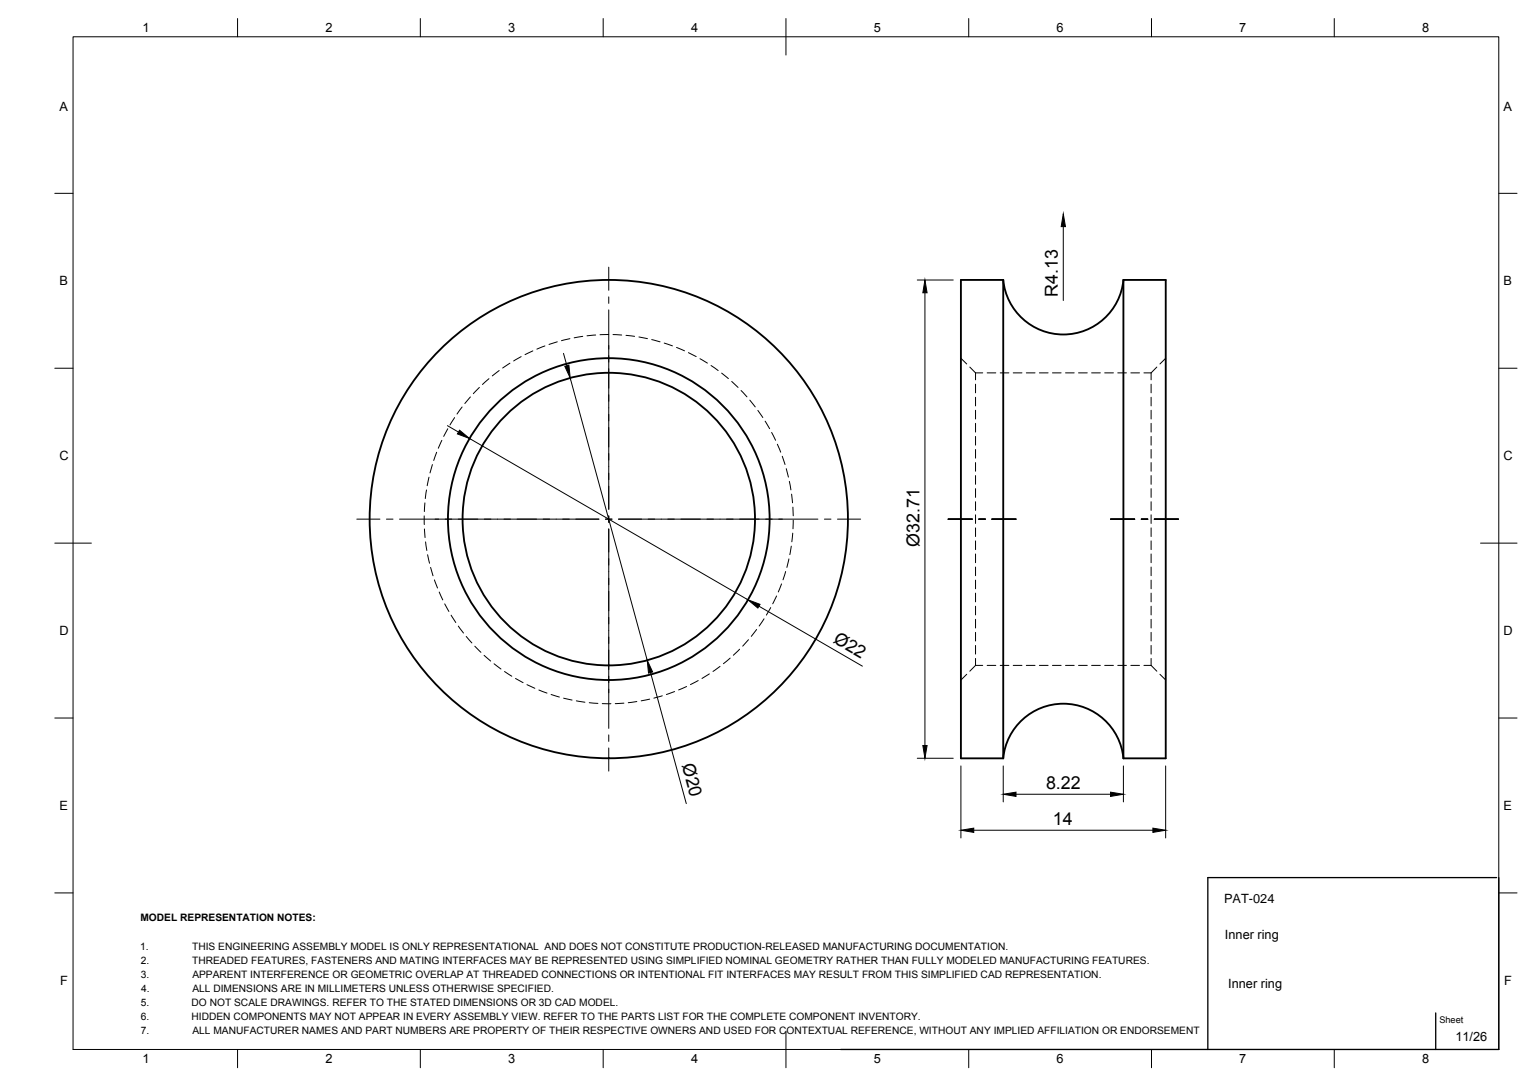
ISO-10303-21;
HEADER;
/* Generated by software containing ST-Developer
 * from STEP Tools, Inc. (www.steptools.com) 
 */

FILE_DESCRIPTION(
/* description */ ('Compact handwheel screw vise'),
/* implementation_level */ '2;1');

FILE_NAME(
/* name */ 'Inner ring.step',
/* time_stamp */ '2026-10-29T16:08:22-07:00',
/* author */ (''),
/* organization */ (''),
/* preprocessor_version */ 'ST-DEVELOPER v20.2',
/* originating_system */ 'Autodesk Translation Framework v15.17.0.0',
/* authorisation */ '');

FILE_SCHEMA (('AUTOMOTIVE_DESIGN { 1 0 10303 214 3 1 1 }'));
ENDSEC;

DATA;
#10=MECHANICAL_DESIGN_GEOMETRIC_PRESENTATION_REPRESENTATION('',(#651),#25074);
#557=TOROIDAL_SURFACE('',#8574,1.675,0.412776);
#562=CONICAL_SURFACE('',#8585,1.05,0.785398163397449);
#563=CONICAL_SURFACE('',#8592,1.05,0.785398163397449);
#595=SHAPE_REPRESENTATION_RELATIONSHIP('SRR','None',#25204,#623);
#623=ADVANCED_BREP_SHAPE_REPRESENTATION('',(#686),#25051);
#651=STYLED_ITEM('',(#25439),#686);
#686=MANIFOLD_SOLID_BREP('Body1',#8060);
#760=FACE_BOUND('',#1628,.T.);
#761=FACE_BOUND('',#1631,.T.);
#879=PLANE('',#8587);
#880=PLANE('',#8590);
#1105=FACE_OUTER_BOUND('',#1623,.T.);
#1106=FACE_OUTER_BOUND('',#1624,.T.);
#1107=FACE_OUTER_BOUND('',#1625,.T.);
#1108=FACE_OUTER_BOUND('',#1626,.T.);
#1109=FACE_OUTER_BOUND('',#1627,.T.);
#1110=FACE_OUTER_BOUND('',#1629,.T.);
#1111=FACE_OUTER_BOUND('',#1630,.T.);
#1112=FACE_OUTER_BOUND('',#1632,.T.);
#1623=EDGE_LOOP('',(#5531,#5532,#5533,#5534,#5535,#5536));
#1624=EDGE_LOOP('',(#5537,#5538,#5539,#5540,#5541));
#1625=EDGE_LOOP('',(#5542,#5543,#5544,#5545));
#1626=EDGE_LOOP('',(#5546,#5547,#5548,#5549));
#1627=EDGE_LOOP('',(#5550));
#1628=EDGE_LOOP('',(#5551));
#1629=EDGE_LOOP('',(#5552,#5553,#5554,#5555,#5556));
#1630=EDGE_LOOP('',(#5557));
#1631=EDGE_LOOP('',(#5558));
#1632=EDGE_LOOP('',(#5559,#5560,#5561,#5562));
#2179=LINE('',#11743,#2687);
#2180=LINE('',#11749,#2688);
#2181=LINE('',#11753,#2689);
#2182=LINE('',#11759,#2690);
#2183=LINE('',#11764,#2691);
#2687=VECTOR('',#9681,1.63531);
#2688=VECTOR('',#9688,1.);
#2689=VECTOR('',#9693,1.05);
#2690=VECTOR('',#9702,1.63531);
#2691=VECTOR('',#9709,1.05);
#3147=CIRCLE('',#8575,1.63531);
#3148=CIRCLE('',#8576,1.63531);
#3149=CIRCLE('',#8577,0.412776);
#3150=CIRCLE('',#8578,1.63531);
#3151=CIRCLE('',#8579,1.63531);
#3152=CIRCLE('',#8581,1.63531);
#3153=CIRCLE('',#8583,1.);
#3154=CIRCLE('',#8584,1.);
#3155=CIRCLE('',#8586,1.1);
#3156=CIRCLE('',#8589,1.63531);
#3157=CIRCLE('',#8591,1.1);
#3456=VERTEX_POINT('',#11732);
#3457=VERTEX_POINT('',#11733);
#3458=VERTEX_POINT('',#11736);
#3459=VERTEX_POINT('',#11738);
#3460=VERTEX_POINT('',#11742);
#3461=VERTEX_POINT('',#11746);
#3462=VERTEX_POINT('',#11748);
#3463=VERTEX_POINT('',#11752);
#3464=VERTEX_POINT('',#11757);
#3465=VERTEX_POINT('',#11761);
#4252=EDGE_CURVE('',#3456,#3457,#3147,.T.);
#4253=EDGE_CURVE('',#3457,#3456,#3148,.T.);
#4254=EDGE_CURVE('',#3457,#3458,#3149,.T.);
#4255=EDGE_CURVE('',#3459,#3458,#3150,.T.);
#4256=EDGE_CURVE('',#3458,#3459,#3151,.T.);
#4257=EDGE_CURVE('',#3459,#3460,#2179,.T.);
#4258=EDGE_CURVE('',#3460,#3460,#3152,.T.);
#4259=EDGE_CURVE('',#3461,#3461,#3153,.T.);
#4260=EDGE_CURVE('',#3461,#3462,#2180,.T.);
#4261=EDGE_CURVE('',#3462,#3462,#3154,.T.);
#4262=EDGE_CURVE('',#3462,#3463,#2181,.T.);
#4263=EDGE_CURVE('',#3463,#3463,#3155,.T.);
#4264=EDGE_CURVE('',#3464,#3464,#3156,.T.);
#4265=EDGE_CURVE('',#3464,#3456,#2182,.T.);
#4266=EDGE_CURVE('',#3465,#3465,#3157,.T.);
#4267=EDGE_CURVE('',#3465,#3461,#2183,.T.);
#5531=ORIENTED_EDGE('',*,*,#4252,.F.);
#5532=ORIENTED_EDGE('',*,*,#4253,.F.);
#5533=ORIENTED_EDGE('',*,*,#4254,.T.);
#5534=ORIENTED_EDGE('',*,*,#4255,.F.);
#5535=ORIENTED_EDGE('',*,*,#4256,.F.);
#5536=ORIENTED_EDGE('',*,*,#4254,.F.);
#5537=ORIENTED_EDGE('',*,*,#4255,.T.);
#5538=ORIENTED_EDGE('',*,*,#4256,.T.);
#5539=ORIENTED_EDGE('',*,*,#4257,.T.);
#5540=ORIENTED_EDGE('',*,*,#4258,.T.);
#5541=ORIENTED_EDGE('',*,*,#4257,.F.);
#5542=ORIENTED_EDGE('',*,*,#4259,.T.);
#5543=ORIENTED_EDGE('',*,*,#4260,.T.);
#5544=ORIENTED_EDGE('',*,*,#4261,.F.);
#5545=ORIENTED_EDGE('',*,*,#4260,.F.);
#5546=ORIENTED_EDGE('',*,*,#4261,.T.);
#5547=ORIENTED_EDGE('',*,*,#4262,.T.);
#5548=ORIENTED_EDGE('',*,*,#4263,.F.);
#5549=ORIENTED_EDGE('',*,*,#4262,.F.);
#5550=ORIENTED_EDGE('',*,*,#4258,.F.);
#5551=ORIENTED_EDGE('',*,*,#4263,.T.);
#5552=ORIENTED_EDGE('',*,*,#4264,.F.);
#5553=ORIENTED_EDGE('',*,*,#4265,.T.);
#5554=ORIENTED_EDGE('',*,*,#4252,.T.);
#5555=ORIENTED_EDGE('',*,*,#4253,.T.);
#5556=ORIENTED_EDGE('',*,*,#4265,.F.);
#5557=ORIENTED_EDGE('',*,*,#4264,.T.);
#5558=ORIENTED_EDGE('',*,*,#4266,.F.);
#5559=ORIENTED_EDGE('',*,*,#4266,.T.);
#5560=ORIENTED_EDGE('',*,*,#4267,.T.);
#5561=ORIENTED_EDGE('',*,*,#4259,.F.);
#5562=ORIENTED_EDGE('',*,*,#4267,.F.);
#7378=CYLINDRICAL_SURFACE('',#8580,1.63531);
#7379=CYLINDRICAL_SURFACE('',#8582,1.);
#7380=CYLINDRICAL_SURFACE('',#8588,1.63531);
#7675=ADVANCED_FACE('',(#1105),#557,.F.);
#7676=ADVANCED_FACE('',(#1106),#7378,.T.);
#7677=ADVANCED_FACE('',(#1107),#7379,.F.);
#7678=ADVANCED_FACE('',(#1108),#562,.F.);
#7679=ADVANCED_FACE('',(#1109,#760),#879,.T.);
#7680=ADVANCED_FACE('',(#1110),#7380,.T.);
#7681=ADVANCED_FACE('',(#1111,#761),#880,.T.);
#7682=ADVANCED_FACE('',(#1112),#563,.F.);
#8060=CLOSED_SHELL('',(#7675,#7676,#7677,#7678,#7679,#7680,#7681,#7682));
#8573=AXIS2_PLACEMENT_3D('',#11730,#9665,#9666);
#8574=AXIS2_PLACEMENT_3D('',#11731,#9667,#9668);
#8575=AXIS2_PLACEMENT_3D('',#11734,#9669,#9670);
#8576=AXIS2_PLACEMENT_3D('',#11735,#9671,#9672);
#8577=AXIS2_PLACEMENT_3D('',#11737,#9673,#9674);
#8578=AXIS2_PLACEMENT_3D('',#11739,#9675,#9676);
#8579=AXIS2_PLACEMENT_3D('',#11740,#9677,#9678);
#8580=AXIS2_PLACEMENT_3D('',#11741,#9679,#9680);
#8581=AXIS2_PLACEMENT_3D('',#11744,#9682,#9683);
#8582=AXIS2_PLACEMENT_3D('',#11745,#9684,#9685);
#8583=AXIS2_PLACEMENT_3D('',#11747,#9686,#9687);
#8584=AXIS2_PLACEMENT_3D('',#11750,#9689,#9690);
#8585=AXIS2_PLACEMENT_3D('',#11751,#9691,#9692);
#8586=AXIS2_PLACEMENT_3D('',#11754,#9694,#9695);
#8587=AXIS2_PLACEMENT_3D('',#11755,#9696,#9697);
#8588=AXIS2_PLACEMENT_3D('',#11756,#9698,#9699);
#8589=AXIS2_PLACEMENT_3D('',#11758,#9700,#9701);
#8590=AXIS2_PLACEMENT_3D('',#11760,#9703,#9704);
#8591=AXIS2_PLACEMENT_3D('',#11762,#9705,#9706);
#8592=AXIS2_PLACEMENT_3D('',#11763,#9707,#9708);
#9665=DIRECTION('axis',(0.,0.,1.));
#9666=DIRECTION('refdir',(1.,0.,0.));
#9667=DIRECTION('center_axis',(0.,-1.,0.));
#9668=DIRECTION('ref_axis',(0.,0.,-1.));
#9669=DIRECTION('center_axis',(0.,-1.,0.));
#9670=DIRECTION('ref_axis',(1.,0.,0.));
#9671=DIRECTION('center_axis',(0.,-1.,0.));
#9672=DIRECTION('ref_axis',(1.,0.,0.));
#9673=DIRECTION('center_axis',(1.,0.,1.22464679914735E-16));
#9674=DIRECTION('ref_axis',(-1.22464679914735E-16,0.,1.));
#9675=DIRECTION('center_axis',(0.,1.,0.));
#9676=DIRECTION('ref_axis',(1.,0.,0.));
#9677=DIRECTION('center_axis',(0.,1.,0.));
#9678=DIRECTION('ref_axis',(1.,0.,0.));
#9679=DIRECTION('center_axis',(0.,-1.,0.));
#9680=DIRECTION('ref_axis',(1.,0.,0.));
#9681=DIRECTION('',(0.,1.,0.));
#9682=DIRECTION('center_axis',(0.,-1.,0.));
#9683=DIRECTION('ref_axis',(1.,0.,0.));
#9684=DIRECTION('center_axis',(0.,-1.,0.));
#9685=DIRECTION('ref_axis',(1.,0.,0.));
#9686=DIRECTION('center_axis',(0.,-1.,0.));
#9687=DIRECTION('ref_axis',(1.,0.,0.));
#9688=DIRECTION('',(0.,1.,0.));
#9689=DIRECTION('center_axis',(0.,-1.,0.));
#9690=DIRECTION('ref_axis',(1.,0.,0.));
#9691=DIRECTION('center_axis',(0.,1.,0.));
#9692=DIRECTION('ref_axis',(1.,0.,0.));
#9693=DIRECTION('',(-0.707106781186548,0.707106781186547,-8.65956056235494E-17));
#9694=DIRECTION('center_axis',(0.,-1.,0.));
#9695=DIRECTION('ref_axis',(1.,0.,0.));
#9696=DIRECTION('center_axis',(0.,1.,0.));
#9697=DIRECTION('ref_axis',(0.,0.,1.));
#9698=DIRECTION('center_axis',(0.,-1.,0.));
#9699=DIRECTION('ref_axis',(1.,0.,0.));
#9700=DIRECTION('center_axis',(0.,-1.,0.));
#9701=DIRECTION('ref_axis',(1.,0.,0.));
#9702=DIRECTION('',(0.,1.,0.));
#9703=DIRECTION('center_axis',(0.,-1.,0.));
#9704=DIRECTION('ref_axis',(0.,0.,-1.));
#9705=DIRECTION('center_axis',(0.,-1.,0.));
#9706=DIRECTION('ref_axis',(1.,0.,0.));
#9707=DIRECTION('center_axis',(0.,-1.,0.));
#9708=DIRECTION('ref_axis',(1.,0.,0.));
#9709=DIRECTION('',(0.707106781186548,0.707106781186547,8.65956056235494E-17));
#11730=CARTESIAN_POINT('',(0.,0.,0.));
#11731=CARTESIAN_POINT('Origin',(0.,0.,0.));
#11732=CARTESIAN_POINT('',(-1.63531,-0.410863395882378,-2.00267715711366E-16));
#11733=CARTESIAN_POINT('',(-2.00267715711366E-16,-0.410863395882378,1.63531));
#11734=CARTESIAN_POINT('Origin',(0.,-0.410863395882378,0.));
#11735=CARTESIAN_POINT('Origin',(0.,-0.410863395882378,0.));
#11736=CARTESIAN_POINT('',(-2.00267715711366E-16,0.410863395882378,1.63531));
#11737=CARTESIAN_POINT('Origin',(-2.05128338857182E-16,0.,1.675));
#11738=CARTESIAN_POINT('',(-1.63531,0.410863395882378,2.00267715711366E-16));
#11739=CARTESIAN_POINT('Origin',(0.,0.410863395882378,0.));
#11740=CARTESIAN_POINT('Origin',(0.,0.410863395882378,0.));
#11741=CARTESIAN_POINT('Origin',(0.,0.,0.));
#11742=CARTESIAN_POINT('',(-1.63531,0.7,-2.00267715711366E-16));
#11743=CARTESIAN_POINT('',(-1.63531,0.,-2.00267715711366E-16));
#11744=CARTESIAN_POINT('Origin',(0.,0.7,0.));
#11745=CARTESIAN_POINT('Origin',(0.,0.,0.));
#11746=CARTESIAN_POINT('',(-1.,-0.6,-1.22464679914735E-16));
#11747=CARTESIAN_POINT('Origin',(0.,-0.6,0.));
#11748=CARTESIAN_POINT('',(-1.,0.6,-1.22464679914735E-16));
#11749=CARTESIAN_POINT('',(-1.,0.,-1.22464679914735E-16));
#11750=CARTESIAN_POINT('Origin',(0.,0.6,0.));
#11751=CARTESIAN_POINT('Origin',(0.,0.65,0.));
#11752=CARTESIAN_POINT('',(-1.1,0.7,-1.34711147906209E-16));
#11753=CARTESIAN_POINT('',(-1.05,0.65,-1.28587913910472E-16));
#11754=CARTESIAN_POINT('Origin',(0.,0.7,0.));
#11755=CARTESIAN_POINT('Origin',(1.63531,0.7,0.));
#11756=CARTESIAN_POINT('Origin',(0.,0.,0.));
#11757=CARTESIAN_POINT('',(-1.63531,-0.7,-2.00267715711366E-16));
#11758=CARTESIAN_POINT('Origin',(0.,-0.7,0.));
#11759=CARTESIAN_POINT('',(-1.63531,0.,-2.00267715711366E-16));
#11760=CARTESIAN_POINT('Origin',(1.1,-0.7,0.));
#11761=CARTESIAN_POINT('',(-1.1,-0.7,-1.34711147906209E-16));
#11762=CARTESIAN_POINT('Origin',(0.,-0.7,0.));
#11763=CARTESIAN_POINT('Origin',(0.,-0.65,0.));
#11764=CARTESIAN_POINT('',(-1.05,-0.65,-1.28587913910472E-16));
#25017=UNCERTAINTY_MEASURE_WITH_UNIT(LENGTH_MEASURE(0.001),#25075,
'DISTANCE_ACCURACY_VALUE',
'Maximum model space distance between geometric entities at asserted c
onnectivities');
#25040=UNCERTAINTY_MEASURE_WITH_UNIT(LENGTH_MEASURE(0.001),#25075,
'DISTANCE_ACCURACY_VALUE',
'Maximum model space distance between geometric entities at asserted c
onnectivities');
#25051=(
GEOMETRIC_REPRESENTATION_CONTEXT(3)
GLOBAL_UNCERTAINTY_ASSIGNED_CONTEXT((#25017))
GLOBAL_UNIT_ASSIGNED_CONTEXT((#25075,#25077,#25078))
REPRESENTATION_CONTEXT('','3D')
);
#25074=(
GEOMETRIC_REPRESENTATION_CONTEXT(3)
GLOBAL_UNCERTAINTY_ASSIGNED_CONTEXT((#25040))
GLOBAL_UNIT_ASSIGNED_CONTEXT((#25075,#25077,#25078))
REPRESENTATION_CONTEXT('','3D')
);
#25075=(
LENGTH_UNIT()
NAMED_UNIT(*)
SI_UNIT(.CENTI.,.METRE.)
);
#25077=(
NAMED_UNIT(*)
PLANE_ANGLE_UNIT()
SI_UNIT($,.RADIAN.)
);
#25078=(
NAMED_UNIT(*)
SI_UNIT($,.STERADIAN.)
SOLID_ANGLE_UNIT()
);
#25089=SHAPE_DEFINITION_REPRESENTATION(#25122,#25204);
#25122=PRODUCT_DEFINITION_SHAPE('',$,#25238);
#25204=SHAPE_REPRESENTATION('',(#8573),#25051);
#25227=PRODUCT_DEFINITION_CONTEXT('part definition',#25328,'design');
#25238=PRODUCT_DEFINITION('Inner ring','Inner ring',#25271,#25227);
#25271=PRODUCT_DEFINITION_FORMATION('',$,#25340);
#25328=APPLICATION_CONTEXT(
'Core Data for Automotive Mechanical Design Process');
#25329=PRODUCT_CONTEXT('part definition',#25328,'mechanical');
#25340=PRODUCT('Inner ring','Inner ring','Inner ring',(#25329));
#25433=COLOUR_RGB('Grey',0.48,0.52,0.57);
#25434=FILL_AREA_STYLE_COLOUR('',#25433);
#25435=FILL_AREA_STYLE('',(#25434));
#25436=SURFACE_STYLE_FILL_AREA(#25435);
#25437=SURFACE_SIDE_STYLE('',(#25436));
#25438=SURFACE_STYLE_USAGE(.BOTH.,#25437);
#25439=PRESENTATION_STYLE_ASSIGNMENT((#25438));
ENDSEC;
END-ISO-10303-21;
